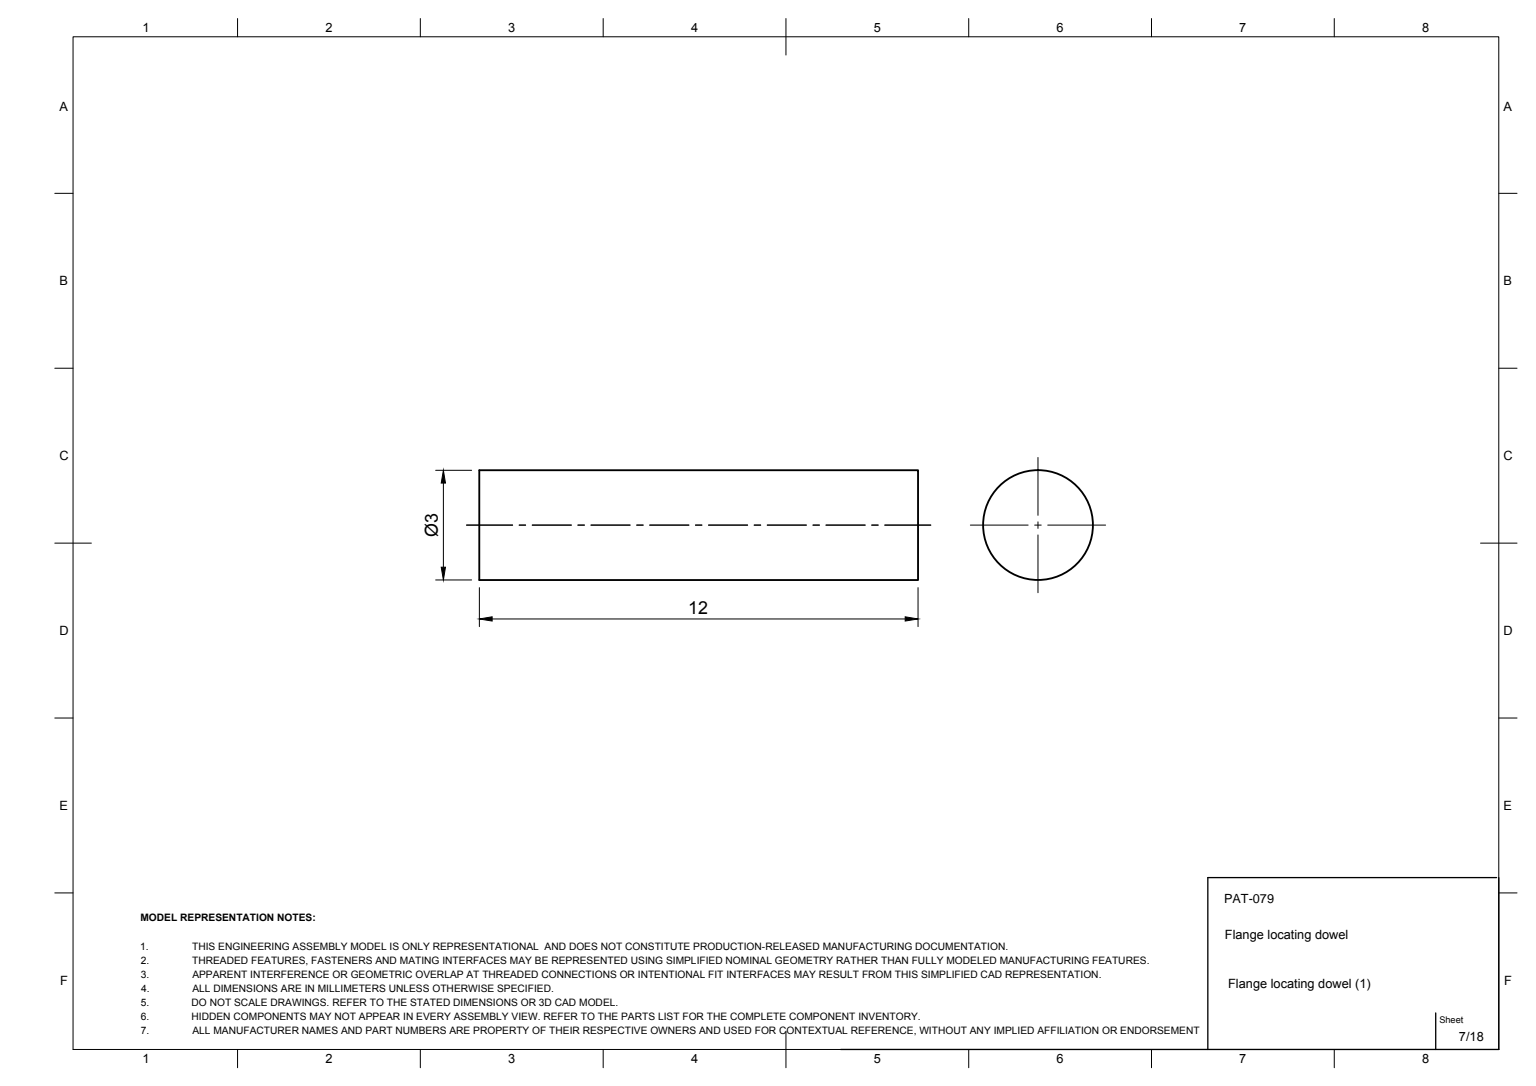
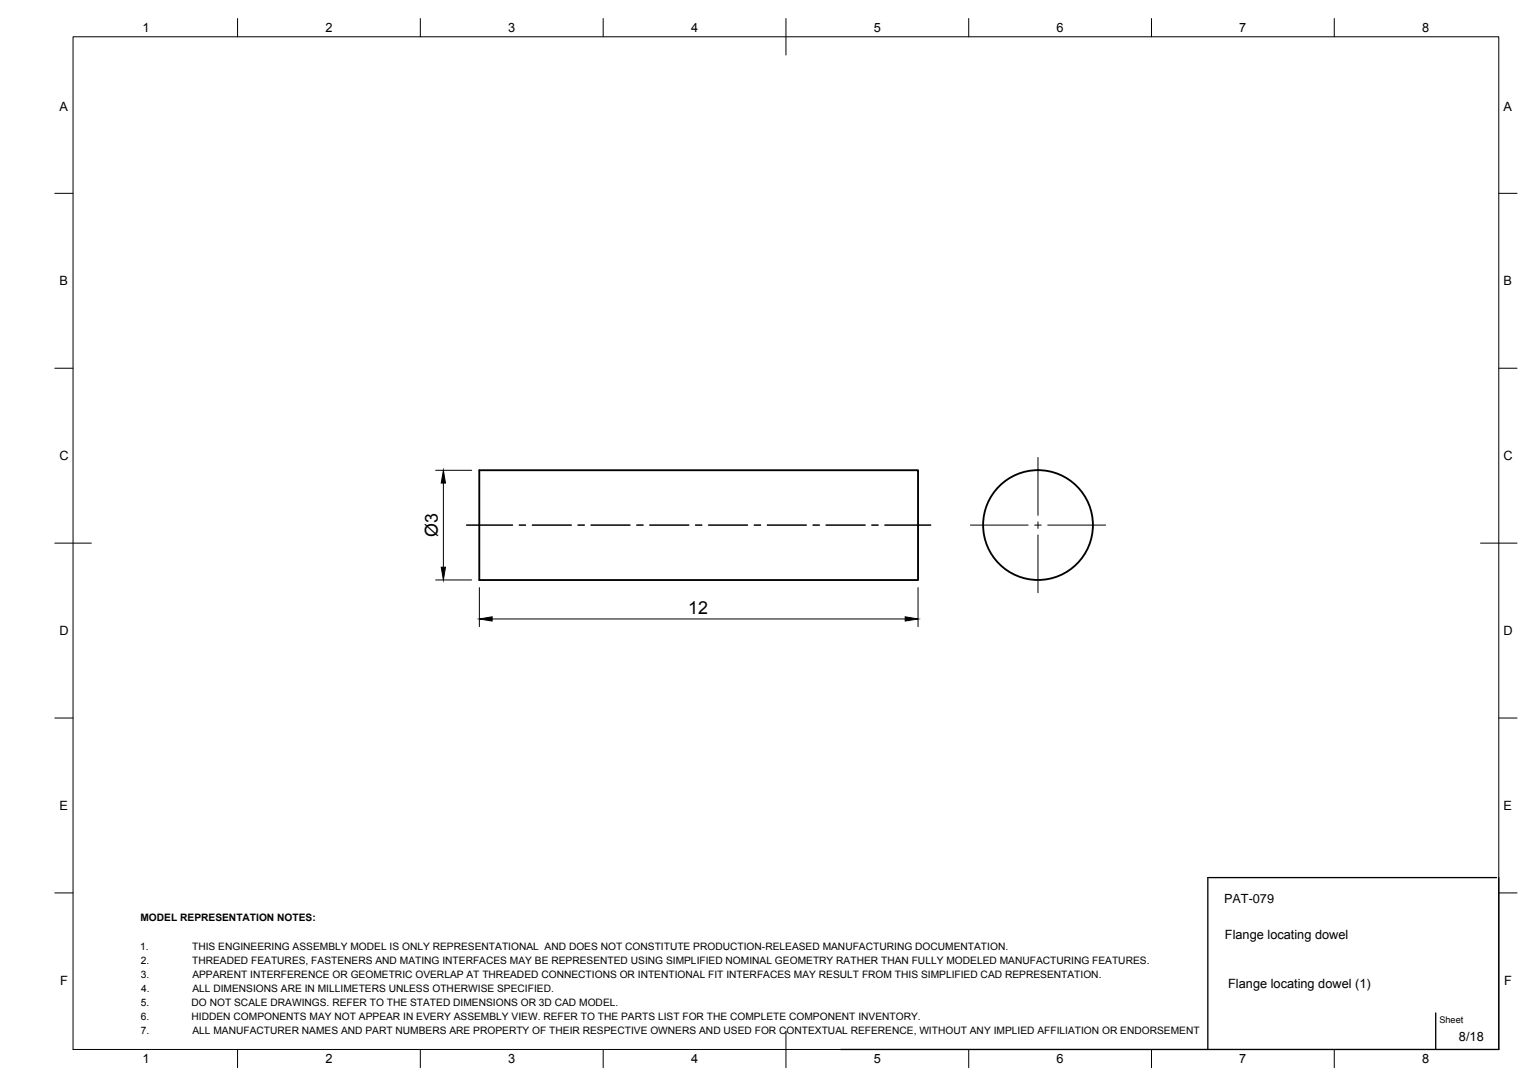
ISO-10303-21;
HEADER;
/* Generated by software containing ST-Developer
 * from STEP Tools, Inc. (www.steptools.com) 
 */

FILE_DESCRIPTION(
/* description */ ('Pipe clamp stand with threaded column'),
/* implementation_level */ '2;1');

FILE_NAME(
/* name */ 'Flange locating dowel.step',
/* time_stamp */ '2026-10-27T10:55:48-07:00',
/* author */ (''),
/* organization */ (''),
/* preprocessor_version */ 'ST-DEVELOPER v20.2',
/* originating_system */ 'Autodesk Translation Framework v15.17.0.0',
/* authorisation */ '');

FILE_SCHEMA (('AUTOMOTIVE_DESIGN { 1 0 10303 214 3 1 1 }'));
ENDSEC;

DATA;
#10=MECHANICAL_DESIGN_GEOMETRIC_PRESENTATION_REPRESENTATION('',(#743),#34433);
#699=SHAPE_REPRESENTATION_RELATIONSHIP('SRR','None',#34541,#721);
#721=ADVANCED_BREP_SHAPE_REPRESENTATION('',(#773),#34409);
#743=STYLED_ITEM('',(#34729),#773);
#773=MANIFOLD_SOLID_BREP('Body1',#8770);
#868=PLANE('',#9295);
#869=PLANE('',#9296);
#1260=FACE_OUTER_BOUND('',#1770,.T.);
#1261=FACE_OUTER_BOUND('',#1771,.T.);
#1262=FACE_OUTER_BOUND('',#1772,.T.);
#1770=EDGE_LOOP('',(#6767,#6768,#6769,#6770));
#1771=EDGE_LOOP('',(#6771));
#1772=EDGE_LOOP('',(#6772));
#2289=LINE('',#28019,#2906);
#2906=VECTOR('',#10440,0.15);
#3340=CIRCLE('',#9293,0.15);
#3341=CIRCLE('',#9294,0.15);
#3862=VERTEX_POINT('',#28016);
#3863=VERTEX_POINT('',#28018);
#4897=EDGE_CURVE('',#3862,#3862,#3340,.T.);
#4898=EDGE_CURVE('',#3862,#3863,#2289,.T.);
#4899=EDGE_CURVE('',#3863,#3863,#3341,.T.);
#6767=ORIENTED_EDGE('',*,*,#4897,.F.);
#6768=ORIENTED_EDGE('',*,*,#4898,.T.);
#6769=ORIENTED_EDGE('',*,*,#4899,.T.);
#6770=ORIENTED_EDGE('',*,*,#4898,.F.);
#6771=ORIENTED_EDGE('',*,*,#4897,.T.);
#6772=ORIENTED_EDGE('',*,*,#4899,.F.);
#8202=CYLINDRICAL_SURFACE('',#9292,0.15);
#8497=ADVANCED_FACE('',(#1260),#8202,.T.);
#8498=ADVANCED_FACE('',(#1261),#868,.T.);
#8499=ADVANCED_FACE('',(#1262),#869,.F.);
#8770=CLOSED_SHELL('',(#8497,#8498,#8499));
#9291=AXIS2_PLACEMENT_3D('',#28014,#10434,#10435);
#9292=AXIS2_PLACEMENT_3D('',#28015,#10436,#10437);
#9293=AXIS2_PLACEMENT_3D('',#28017,#10438,#10439);
#9294=AXIS2_PLACEMENT_3D('',#28020,#10441,#10442);
#9295=AXIS2_PLACEMENT_3D('',#28021,#10443,#10444);
#9296=AXIS2_PLACEMENT_3D('',#28022,#10445,#10446);
#10434=DIRECTION('axis',(0.,0.,1.));
#10435=DIRECTION('refdir',(1.,0.,0.));
#10436=DIRECTION('center_axis',(0.,0.,1.));
#10437=DIRECTION('ref_axis',(1.,0.,0.));
#10438=DIRECTION('center_axis',(0.,0.,1.));
#10439=DIRECTION('ref_axis',(1.,0.,0.));
#10440=DIRECTION('',(0.,0.,-1.));
#10441=DIRECTION('center_axis',(0.,0.,1.));
#10442=DIRECTION('ref_axis',(1.,0.,0.));
#10443=DIRECTION('center_axis',(0.,0.,1.));
#10444=DIRECTION('ref_axis',(1.,0.,0.));
#10445=DIRECTION('center_axis',(0.,0.,1.));
#10446=DIRECTION('ref_axis',(1.,0.,0.));
#28014=CARTESIAN_POINT('',(0.,0.,0.));
#28015=CARTESIAN_POINT('Origin',(-10.7,1.5,0.6));
#28016=CARTESIAN_POINT('',(-10.85,1.5,1.8));
#28017=CARTESIAN_POINT('Origin',(-10.7,1.5,1.8));
#28018=CARTESIAN_POINT('',(-10.85,1.5,0.6));
#28019=CARTESIAN_POINT('',(-10.85,1.5,0.6));
#28020=CARTESIAN_POINT('Origin',(-10.7,1.5,0.6));
#28021=CARTESIAN_POINT('Origin',(-10.7,1.5,1.8));
#28022=CARTESIAN_POINT('Origin',(-10.7,1.5,0.6));
#34380=UNCERTAINTY_MEASURE_WITH_UNIT(LENGTH_MEASURE(0.001),#34434,
'DISTANCE_ACCURACY_VALUE',
'Maximum model space distance between geometric entities at asserted c
onnectivities');
#34404=UNCERTAINTY_MEASURE_WITH_UNIT(LENGTH_MEASURE(0.001),#34434,
'DISTANCE_ACCURACY_VALUE',
'Maximum model space distance between geometric entities at asserted c
onnectivities');
#34409=(
GEOMETRIC_REPRESENTATION_CONTEXT(3)
GLOBAL_UNCERTAINTY_ASSIGNED_CONTEXT((#34380))
GLOBAL_UNIT_ASSIGNED_CONTEXT((#34434,#34436,#34437))
REPRESENTATION_CONTEXT('','3D')
);
#34433=(
GEOMETRIC_REPRESENTATION_CONTEXT(3)
GLOBAL_UNCERTAINTY_ASSIGNED_CONTEXT((#34404))
GLOBAL_UNIT_ASSIGNED_CONTEXT((#34434,#34436,#34437))
REPRESENTATION_CONTEXT('','3D')
);
#34434=(
LENGTH_UNIT()
NAMED_UNIT(*)
SI_UNIT(.CENTI.,.METRE.)
);
#34436=(
NAMED_UNIT(*)
PLANE_ANGLE_UNIT()
SI_UNIT($,.RADIAN.)
);
#34437=(
NAMED_UNIT(*)
SI_UNIT($,.STERADIAN.)
SOLID_ANGLE_UNIT()
);
#34442=SHAPE_DEFINITION_REPRESENTATION(#34470,#34541);
#34470=PRODUCT_DEFINITION_SHAPE('',$,#34570);
#34541=SHAPE_REPRESENTATION('',(#9291),#34409);
#34565=PRODUCT_DEFINITION_CONTEXT('part definition',#34651,'design');
#34570=PRODUCT_DEFINITION('Flange locating dowel',
'Flange locating dowel',#34598,#34565);
#34598=PRODUCT_DEFINITION_FORMATION('',$,#34657);
#34651=APPLICATION_CONTEXT(
'Core Data for Automotive Mechanical Design Process');
#34652=PRODUCT_CONTEXT('part definition',#34651,'mechanical');
#34657=PRODUCT('Flange locating dowel','Flange locating dowel',
'Flange locating dowel',(#34652));
#34723=COLOUR_RGB('Light Blue',0.38,0.62,0.78);
#34724=FILL_AREA_STYLE_COLOUR('',#34723);
#34725=FILL_AREA_STYLE('',(#34724));
#34726=SURFACE_STYLE_FILL_AREA(#34725);
#34727=SURFACE_SIDE_STYLE('',(#34726));
#34728=SURFACE_STYLE_USAGE(.BOTH.,#34727);
#34729=PRESENTATION_STYLE_ASSIGNMENT((#34728));
ENDSEC;
END-ISO-10303-21;
